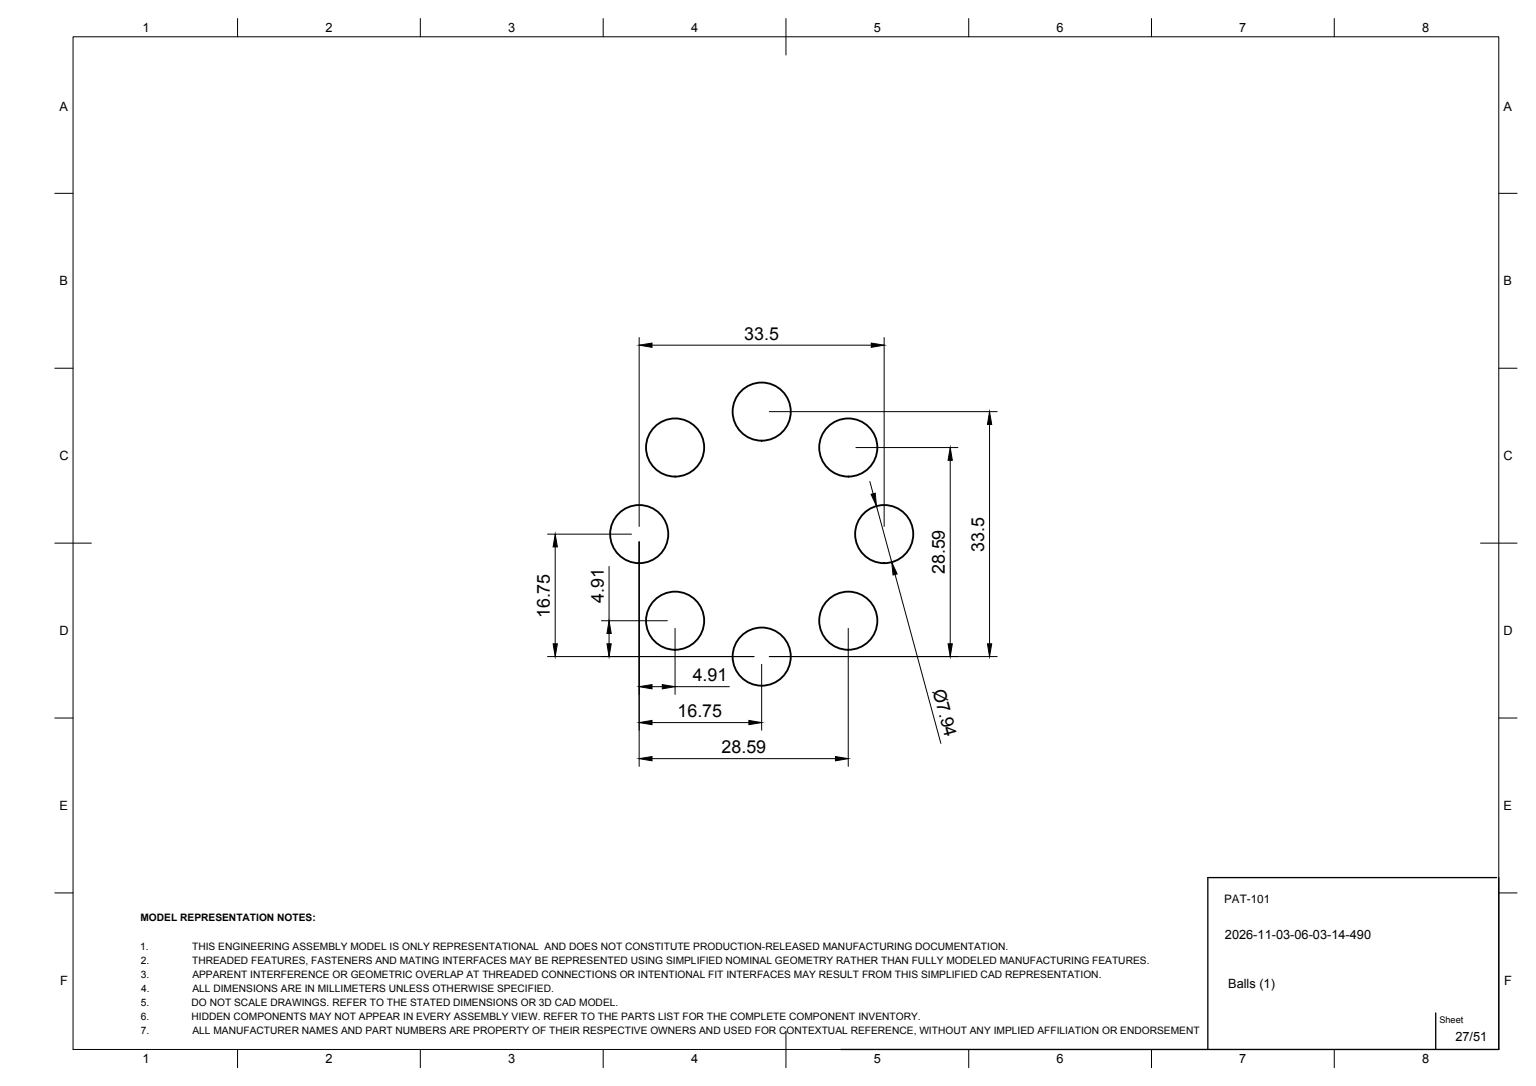
ISO-10303-21;
HEADER;
/* Generated by software containing ST-Developer
 * from STEP Tools, Inc. (www.steptools.com) 
 */

FILE_DESCRIPTION(
/* description */ ('Spur gear reduction stage 2-1 on bearing plates'),
/* implementation_level */ '2;1');

FILE_NAME(
/* name */ 'Balls (1).step',
/* time_stamp */ '2026-10-28T03:22:07-07:00',
/* author */ (''),
/* organization */ (''),
/* preprocessor_version */ 'ST-DEVELOPER v20.2',
/* originating_system */ 'Autodesk Translation Framework v15.17.0.0',
/* authorisation */ '');

FILE_SCHEMA (('AUTOMOTIVE_DESIGN { 1 0 10303 214 3 1 1 }'));
ENDSEC;

DATA;
#10=MECHANICAL_DESIGN_GEOMETRIC_PRESENTATION_REPRESENTATION('',(#974,#975,#976,#977,#978,#979,#980,#981),#53909);
#809=SPHERICAL_SURFACE('',#12323,0.3969);
#810=SPHERICAL_SURFACE('',#12325,0.3969);
#811=SPHERICAL_SURFACE('',#12327,0.3969);
#812=SPHERICAL_SURFACE('',#12329,0.3969);
#813=SPHERICAL_SURFACE('',#12331,0.3969);
#814=SPHERICAL_SURFACE('',#12333,0.3969);
#815=SPHERICAL_SURFACE('',#12335,0.3969);
#816=SPHERICAL_SURFACE('',#12337,0.3969);
#881=SHAPE_REPRESENTATION_RELATIONSHIP('SRR','None',#54110,#924);
#924=ADVANCED_BREP_SHAPE_REPRESENTATION('',(#1030,#1031,#1032,#1033,#1034,
#1035,#1036,#1037),#53884);
#974=STYLED_ITEM('',(#54397),#1030);
#975=STYLED_ITEM('',(#54397),#1031);
#976=STYLED_ITEM('',(#54397),#1032);
#977=STYLED_ITEM('',(#54397),#1033);
#978=STYLED_ITEM('',(#54397),#1034);
#979=STYLED_ITEM('',(#54397),#1035);
#980=STYLED_ITEM('',(#54397),#1036);
#981=STYLED_ITEM('',(#54397),#1037);
#1030=MANIFOLD_SOLID_BREP('Body1',#11300);
#1031=MANIFOLD_SOLID_BREP('Body2',#11301);
#1032=MANIFOLD_SOLID_BREP('Body3',#11302);
#1033=MANIFOLD_SOLID_BREP('Body4',#11303);
#1034=MANIFOLD_SOLID_BREP('Body5',#11304);
#1035=MANIFOLD_SOLID_BREP('Body6',#11305);
#1036=MANIFOLD_SOLID_BREP('Body7',#11306);
#1037=MANIFOLD_SOLID_BREP('Body8',#11307);
#1731=FACE_OUTER_BOUND('',#2510,.T.);
#1732=FACE_OUTER_BOUND('',#2511,.T.);
#1733=FACE_OUTER_BOUND('',#2512,.T.);
#1734=FACE_OUTER_BOUND('',#2513,.T.);
#1735=FACE_OUTER_BOUND('',#2514,.T.);
#1736=FACE_OUTER_BOUND('',#2515,.T.);
#1737=FACE_OUTER_BOUND('',#2516,.T.);
#1738=FACE_OUTER_BOUND('',#2517,.T.);
#2510=EDGE_LOOP('',(#8270,#8271));
#2511=EDGE_LOOP('',(#8272,#8273));
#2512=EDGE_LOOP('',(#8274,#8275));
#2513=EDGE_LOOP('',(#8276,#8277));
#2514=EDGE_LOOP('',(#8278,#8279));
#2515=EDGE_LOOP('',(#8280,#8281));
#2516=EDGE_LOOP('',(#8282,#8283));
#2517=EDGE_LOOP('',(#8284,#8285));
#4518=CIRCLE('',#12324,0.3969);
#4519=CIRCLE('',#12326,0.3969);
#4520=CIRCLE('',#12328,0.3969);
#4521=CIRCLE('',#12330,0.3969);
#4522=CIRCLE('',#12332,0.3969);
#4523=CIRCLE('',#12334,0.3969);
#4524=CIRCLE('',#12336,0.3969);
#4525=CIRCLE('',#12338,0.3969);
#5094=VERTEX_POINT('',#17297);
#5095=VERTEX_POINT('',#17298);
#5096=VERTEX_POINT('',#17301);
#5097=VERTEX_POINT('',#17302);
#5098=VERTEX_POINT('',#17305);
#5099=VERTEX_POINT('',#17306);
#5100=VERTEX_POINT('',#17309);
#5101=VERTEX_POINT('',#17310);
#5102=VERTEX_POINT('',#17313);
#5103=VERTEX_POINT('',#17314);
#5104=VERTEX_POINT('',#17317);
#5105=VERTEX_POINT('',#17318);
#5106=VERTEX_POINT('',#17321);
#5107=VERTEX_POINT('',#17322);
#5108=VERTEX_POINT('',#17325);
#5109=VERTEX_POINT('',#17326);
#6277=EDGE_CURVE('',#5094,#5095,#4518,.T.);
#6278=EDGE_CURVE('',#5096,#5097,#4519,.T.);
#6279=EDGE_CURVE('',#5098,#5099,#4520,.T.);
#6280=EDGE_CURVE('',#5100,#5101,#4521,.T.);
#6281=EDGE_CURVE('',#5102,#5103,#4522,.T.);
#6282=EDGE_CURVE('',#5104,#5105,#4523,.T.);
#6283=EDGE_CURVE('',#5106,#5107,#4524,.T.);
#6284=EDGE_CURVE('',#5108,#5109,#4525,.T.);
#8270=ORIENTED_EDGE('',*,*,#6277,.T.);
#8271=ORIENTED_EDGE('',*,*,#6277,.F.);
#8272=ORIENTED_EDGE('',*,*,#6278,.T.);
#8273=ORIENTED_EDGE('',*,*,#6278,.F.);
#8274=ORIENTED_EDGE('',*,*,#6279,.T.);
#8275=ORIENTED_EDGE('',*,*,#6279,.F.);
#8276=ORIENTED_EDGE('',*,*,#6280,.T.);
#8277=ORIENTED_EDGE('',*,*,#6280,.F.);
#8278=ORIENTED_EDGE('',*,*,#6281,.T.);
#8279=ORIENTED_EDGE('',*,*,#6281,.F.);
#8280=ORIENTED_EDGE('',*,*,#6282,.T.);
#8281=ORIENTED_EDGE('',*,*,#6282,.F.);
#8282=ORIENTED_EDGE('',*,*,#6283,.T.);
#8283=ORIENTED_EDGE('',*,*,#6283,.F.);
#8284=ORIENTED_EDGE('',*,*,#6284,.T.);
#8285=ORIENTED_EDGE('',*,*,#6284,.F.);
#10851=ADVANCED_FACE('',(#1731),#809,.T.);
#10852=ADVANCED_FACE('',(#1732),#810,.T.);
#10853=ADVANCED_FACE('',(#1733),#811,.T.);
#10854=ADVANCED_FACE('',(#1734),#812,.T.);
#10855=ADVANCED_FACE('',(#1735),#813,.T.);
#10856=ADVANCED_FACE('',(#1736),#814,.T.);
#10857=ADVANCED_FACE('',(#1737),#815,.T.);
#10858=ADVANCED_FACE('',(#1738),#816,.T.);
#11300=CLOSED_SHELL('',(#10851));
#11301=CLOSED_SHELL('',(#10852));
#11302=CLOSED_SHELL('',(#10853));
#11303=CLOSED_SHELL('',(#10854));
#11304=CLOSED_SHELL('',(#10855));
#11305=CLOSED_SHELL('',(#10856));
#11306=CLOSED_SHELL('',(#10857));
#11307=CLOSED_SHELL('',(#10858));
#12322=AXIS2_PLACEMENT_3D('',#17295,#14200,#14201);
#12323=AXIS2_PLACEMENT_3D('',#17296,#14202,#14203);
#12324=AXIS2_PLACEMENT_3D('',#17299,#14204,#14205);
#12325=AXIS2_PLACEMENT_3D('',#17300,#14206,#14207);
#12326=AXIS2_PLACEMENT_3D('',#17303,#14208,#14209);
#12327=AXIS2_PLACEMENT_3D('',#17304,#14210,#14211);
#12328=AXIS2_PLACEMENT_3D('',#17307,#14212,#14213);
#12329=AXIS2_PLACEMENT_3D('',#17308,#14214,#14215);
#12330=AXIS2_PLACEMENT_3D('',#17311,#14216,#14217);
#12331=AXIS2_PLACEMENT_3D('',#17312,#14218,#14219);
#12332=AXIS2_PLACEMENT_3D('',#17315,#14220,#14221);
#12333=AXIS2_PLACEMENT_3D('',#17316,#14222,#14223);
#12334=AXIS2_PLACEMENT_3D('',#17319,#14224,#14225);
#12335=AXIS2_PLACEMENT_3D('',#17320,#14226,#14227);
#12336=AXIS2_PLACEMENT_3D('',#17323,#14228,#14229);
#12337=AXIS2_PLACEMENT_3D('',#17324,#14230,#14231);
#12338=AXIS2_PLACEMENT_3D('',#17327,#14232,#14233);
#14200=DIRECTION('axis',(0.,0.,1.));
#14201=DIRECTION('refdir',(1.,0.,0.));
#14202=DIRECTION('center_axis',(0.,0.,1.));
#14203=DIRECTION('ref_axis',(1.,0.,0.));
#14204=DIRECTION('center_axis',(1.22464679914735E-16,-1.,0.));
#14205=DIRECTION('ref_axis',(-1.,-1.22464679914735E-16,0.));
#14206=DIRECTION('center_axis',(0.707106781186548,0.,0.707106781186548));
#14207=DIRECTION('ref_axis',(0.707106781186548,0.,-0.707106781186548));
#14208=DIRECTION('center_axis',(8.65956056235493E-17,-1.,-8.65956056235493E-17));
#14209=DIRECTION('ref_axis',(-0.707106781186548,-1.22464679914735E-16,0.707106781186548));
#14210=DIRECTION('center_axis',(1.,0.,0.));
#14211=DIRECTION('ref_axis',(6.12323399573677E-17,0.,-1.));
#14212=DIRECTION('center_axis',(7.49879891330929E-33,-1.,-1.22464679914735E-16));
#14213=DIRECTION('ref_axis',(-6.12323399573677E-17,-1.22464679914735E-16,
1.));
#14214=DIRECTION('center_axis',(0.707106781186548,0.,-0.707106781186548));
#14215=DIRECTION('ref_axis',(-0.707106781186548,0.,-0.707106781186548));
#14216=DIRECTION('center_axis',(-8.65956056235493E-17,-1.,-8.65956056235493E-17));
#14217=DIRECTION('ref_axis',(0.707106781186548,-1.22464679914735E-16,0.707106781186548));
#14218=DIRECTION('center_axis',(0.,0.,-1.));
#14219=DIRECTION('ref_axis',(-1.,0.,-1.22464679914735E-16));
#14220=DIRECTION('center_axis',(-1.22464679914735E-16,-1.,-1.49975978266186E-32));
#14221=DIRECTION('ref_axis',(1.,-1.22464679914735E-16,1.22464679914735E-16));
#14222=DIRECTION('center_axis',(-0.707106781186548,0.,-0.707106781186548));
#14223=DIRECTION('ref_axis',(-0.707106781186548,0.,0.707106781186548));
#14224=DIRECTION('center_axis',(-8.65956056235493E-17,-1.,8.65956056235493E-17));
#14225=DIRECTION('ref_axis',(0.707106781186548,-1.22464679914735E-16,-0.707106781186548));
#14226=DIRECTION('center_axis',(-1.,0.,0.));
#14227=DIRECTION('ref_axis',(-1.83697019872103E-16,0.,1.));
#14228=DIRECTION('center_axis',(-2.24963967399279E-32,-1.,1.22464679914735E-16));
#14229=DIRECTION('ref_axis',(1.83697019872103E-16,-1.22464679914735E-16,
-1.));
#14230=DIRECTION('center_axis',(-0.707106781186548,0.,0.707106781186548));
#14231=DIRECTION('ref_axis',(0.707106781186548,0.,0.707106781186548));
#14232=DIRECTION('center_axis',(8.65956056235493E-17,-1.,8.65956056235494E-17));
#14233=DIRECTION('ref_axis',(-0.707106781186548,-1.22464679914735E-16,-0.707106781186548));
#17295=CARTESIAN_POINT('',(0.,0.,0.));
#17296=CARTESIAN_POINT('Origin',(1.675,0.,0.));
#17297=CARTESIAN_POINT('',(1.675,-2.97627328869245E-33,0.3969));
#17298=CARTESIAN_POINT('',(1.675,-2.97627328869245E-33,-0.3969));
#17299=CARTESIAN_POINT('Origin',(1.675,0.,0.));
#17300=CARTESIAN_POINT('Origin',(1.18440385848747,0.,-1.18440385848747));
#17301=CARTESIAN_POINT('',(1.46505453994041,3.1867025333467E-33,-0.903753177034526));
#17302=CARTESIAN_POINT('',(0.903753177034527,-9.13924911073161E-33,-1.46505453994041));
#17303=CARTESIAN_POINT('Origin',(1.18440385848747,0.,-1.18440385848747));
#17304=CARTESIAN_POINT('Origin',(1.02564169428591E-16,0.,-1.675));
#17305=CARTESIAN_POINT('',(0.3969,-2.97627328869246E-33,-1.675));
#17306=CARTESIAN_POINT('',(-0.3969,-2.97627328869245E-33,-1.675));
#17307=CARTESIAN_POINT('Origin',(1.02564169428591E-16,0.,-1.675));
#17308=CARTESIAN_POINT('Origin',(-1.18440385848747,0.,-1.18440385848747));
#17309=CARTESIAN_POINT('',(-0.903753177034526,3.1867025333467E-33,-1.46505453994041));
#17310=CARTESIAN_POINT('',(-1.46505453994041,-9.13924911073161E-33,-0.903753177034527));
#17311=CARTESIAN_POINT('Origin',(-1.18440385848747,0.,-1.18440385848747));
#17312=CARTESIAN_POINT('Origin',(-1.675,0.,-2.05128338857182E-16));
#17313=CARTESIAN_POINT('',(-1.675,-2.97627328869246E-33,-0.3969));
#17314=CARTESIAN_POINT('',(-1.675,-2.97627328869245E-33,0.3969));
#17315=CARTESIAN_POINT('Origin',(-1.675,0.,-2.05128338857182E-16));
#17316=CARTESIAN_POINT('Origin',(-1.18440385848747,0.,1.18440385848747));
#17317=CARTESIAN_POINT('',(-1.46505453994041,6.26819044436628E-33,0.903753177034526));
#17318=CARTESIAN_POINT('',(-0.903753177034527,-1.22207370217512E-32,1.46505453994041));
#17319=CARTESIAN_POINT('Origin',(-1.18440385848747,0.,1.18440385848747));
#17320=CARTESIAN_POINT('Origin',(-3.07692508285772E-16,0.,1.675));
#17321=CARTESIAN_POINT('',(-0.3969,-2.97627328869246E-33,1.675));
#17322=CARTESIAN_POINT('',(0.396899999999999,-2.97627328869245E-33,1.675));
#17323=CARTESIAN_POINT('Origin',(-3.07692508285772E-16,0.,1.675));
#17324=CARTESIAN_POINT('Origin',(1.18440385848747,0.,1.18440385848747));
#17325=CARTESIAN_POINT('',(0.903753177034526,9.34967835538585E-33,1.46505453994041));
#17326=CARTESIAN_POINT('',(1.46505453994041,-1.53022249327708E-32,0.903753177034527));
#17327=CARTESIAN_POINT('Origin',(1.18440385848747,0.,1.18440385848747));
#53834=UNCERTAINTY_MEASURE_WITH_UNIT(LENGTH_MEASURE(0.001),#53910,
'DISTANCE_ACCURACY_VALUE',
'Maximum model space distance between geometric entities at asserted c
onnectivities');
#53859=UNCERTAINTY_MEASURE_WITH_UNIT(LENGTH_MEASURE(0.001),#53910,
'DISTANCE_ACCURACY_VALUE',
'Maximum model space distance between geometric entities at asserted c
onnectivities');
#53884=(
GEOMETRIC_REPRESENTATION_CONTEXT(3)
GLOBAL_UNCERTAINTY_ASSIGNED_CONTEXT((#53834))
GLOBAL_UNIT_ASSIGNED_CONTEXT((#53910,#53912,#53913))
REPRESENTATION_CONTEXT('','3D')
);
#53909=(
GEOMETRIC_REPRESENTATION_CONTEXT(3)
GLOBAL_UNCERTAINTY_ASSIGNED_CONTEXT((#53859))
GLOBAL_UNIT_ASSIGNED_CONTEXT((#53910,#53912,#53913))
REPRESENTATION_CONTEXT('','3D')
);
#53910=(
LENGTH_UNIT()
NAMED_UNIT(*)
SI_UNIT(.CENTI.,.METRE.)
);
#53912=(
NAMED_UNIT(*)
PLANE_ANGLE_UNIT()
SI_UNIT($,.RADIAN.)
);
#53913=(
NAMED_UNIT(*)
SI_UNIT($,.STERADIAN.)
SOLID_ANGLE_UNIT()
);
#53938=SHAPE_DEFINITION_REPRESENTATION(#53992,#54110);
#53992=PRODUCT_DEFINITION_SHAPE('',$,#54160);
#54110=SHAPE_REPRESENTATION('',(#12322),#53884);
#54135=PRODUCT_DEFINITION_CONTEXT('part definition',#54284,'design');
#54160=PRODUCT_DEFINITION('Balls (1)','Balls (1)',#54209,#54135);
#54209=PRODUCT_DEFINITION_FORMATION('',$,#54310);
#54284=APPLICATION_CONTEXT(
'Core Data for Automotive Mechanical Design Process');
#54285=PRODUCT_CONTEXT('part definition',#54284,'mechanical');
#54310=PRODUCT('Balls (1)','Balls (1)','Balls (1)',(#54285));
#54391=COLOUR_RGB('Grey',0.48,0.52,0.57);
#54392=FILL_AREA_STYLE_COLOUR('',#54391);
#54393=FILL_AREA_STYLE('',(#54392));
#54394=SURFACE_STYLE_FILL_AREA(#54393);
#54395=SURFACE_SIDE_STYLE('',(#54394));
#54396=SURFACE_STYLE_USAGE(.BOTH.,#54395);
#54397=PRESENTATION_STYLE_ASSIGNMENT((#54396));
ENDSEC;
END-ISO-10303-21;
